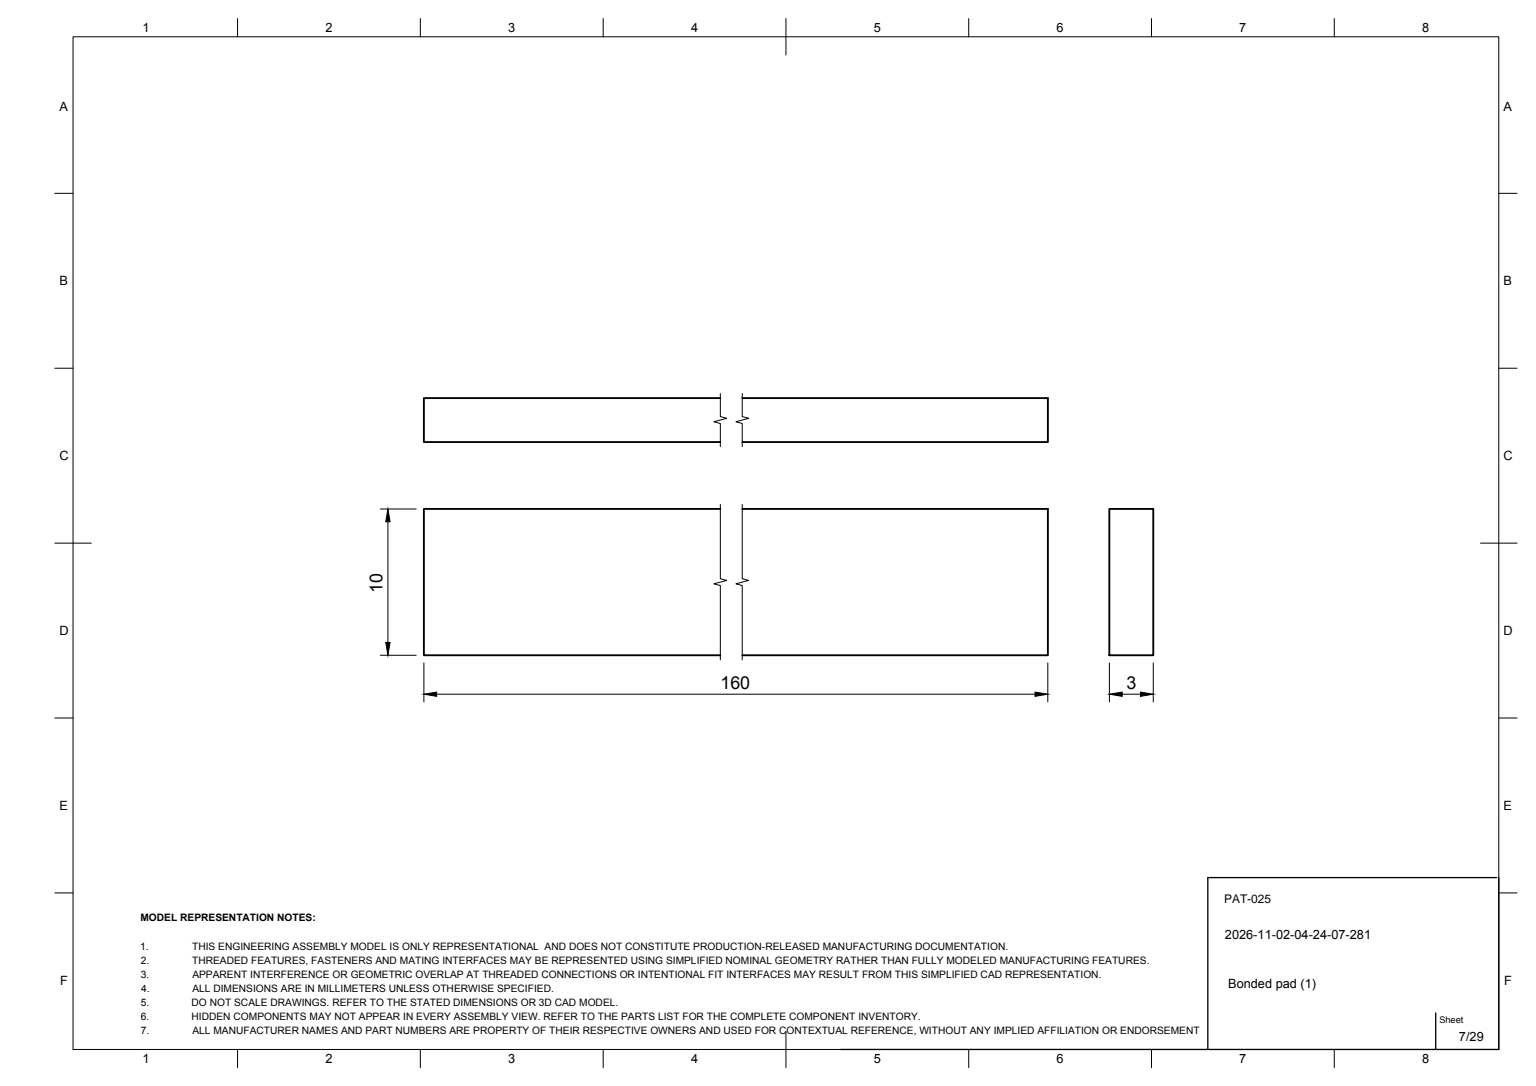
ISO-10303-21;
HEADER;
/* Generated by software containing ST-Developer
 * from STEP Tools, Inc. (www.steptools.com) 
 */

FILE_DESCRIPTION(
/* description */ ('Counter shaft with two pulleys and keyed hub'),
/* implementation_level */ '2;1');

FILE_NAME(
/* name */ 'Bonded pad (1).step',
/* time_stamp */ '2026-10-27T10:46:10-07:00',
/* author */ (''),
/* organization */ (''),
/* preprocessor_version */ 'ST-DEVELOPER v20.2',
/* originating_system */ 'Autodesk Translation Framework v15.17.0.0',
/* authorisation */ '');

FILE_SCHEMA (('AUTOMOTIVE_DESIGN { 1 0 10303 214 3 1 1 }'));
ENDSEC;

DATA;
#10=MECHANICAL_DESIGN_GEOMETRIC_PRESENTATION_REPRESENTATION('',(#292),#10821);
#242=SHAPE_REPRESENTATION_RELATIONSHIP('SRR','None',#10928,#267);
#267=ADVANCED_BREP_SHAPE_REPRESENTATION('',(#318),#10796);
#292=STYLED_ITEM('',(#11149),#318);
#318=MANIFOLD_SOLID_BREP('Body1',#5575);
#443=PLANE('',#5906);
#444=PLANE('',#5907);
#445=PLANE('',#5908);
#446=PLANE('',#5909);
#447=PLANE('',#5910);
#448=PLANE('',#5911);
#604=FACE_OUTER_BOUND('',#926,.T.);
#605=FACE_OUTER_BOUND('',#927,.T.);
#606=FACE_OUTER_BOUND('',#928,.T.);
#607=FACE_OUTER_BOUND('',#929,.T.);
#608=FACE_OUTER_BOUND('',#930,.T.);
#609=FACE_OUTER_BOUND('',#931,.T.);
#926=EDGE_LOOP('',(#3701,#3702,#3703,#3704));
#927=EDGE_LOOP('',(#3705,#3706,#3707,#3708));
#928=EDGE_LOOP('',(#3709,#3710,#3711,#3712));
#929=EDGE_LOOP('',(#3713,#3714,#3715,#3716));
#930=EDGE_LOOP('',(#3717,#3718,#3719,#3720));
#931=EDGE_LOOP('',(#3721,#3722,#3723,#3724));
#1335=LINE('',#8396,#1724);
#1336=LINE('',#8398,#1725);
#1337=LINE('',#8400,#1726);
#1338=LINE('',#8401,#1727);
#1339=LINE('',#8404,#1728);
#1340=LINE('',#8406,#1729);
#1341=LINE('',#8407,#1730);
#1342=LINE('',#8410,#1731);
#1343=LINE('',#8412,#1732);
#1344=LINE('',#8413,#1733);
#1345=LINE('',#8415,#1734);
#1346=LINE('',#8416,#1735);
#1724=VECTOR('',#6647,1.);
#1725=VECTOR('',#6648,1.);
#1726=VECTOR('',#6649,1.);
#1727=VECTOR('',#6650,1.);
#1728=VECTOR('',#6653,1.);
#1729=VECTOR('',#6654,1.);
#1730=VECTOR('',#6655,1.);
#1731=VECTOR('',#6658,1.);
#1732=VECTOR('',#6659,1.);
#1733=VECTOR('',#6660,1.);
#1734=VECTOR('',#6663,1.);
#1735=VECTOR('',#6664,1.);
#2408=VERTEX_POINT('',#8394);
#2409=VERTEX_POINT('',#8395);
#2410=VERTEX_POINT('',#8397);
#2411=VERTEX_POINT('',#8399);
#2412=VERTEX_POINT('',#8403);
#2413=VERTEX_POINT('',#8405);
#2414=VERTEX_POINT('',#8409);
#2415=VERTEX_POINT('',#8411);
#2923=EDGE_CURVE('',#2408,#2409,#1335,.T.);
#2924=EDGE_CURVE('',#2409,#2410,#1336,.T.);
#2925=EDGE_CURVE('',#2411,#2410,#1337,.T.);
#2926=EDGE_CURVE('',#2408,#2411,#1338,.T.);
#2927=EDGE_CURVE('',#2412,#2408,#1339,.T.);
#2928=EDGE_CURVE('',#2413,#2411,#1340,.T.);
#2929=EDGE_CURVE('',#2412,#2413,#1341,.T.);
#2930=EDGE_CURVE('',#2414,#2412,#1342,.T.);
#2931=EDGE_CURVE('',#2415,#2413,#1343,.T.);
#2932=EDGE_CURVE('',#2414,#2415,#1344,.T.);
#2933=EDGE_CURVE('',#2409,#2414,#1345,.T.);
#2934=EDGE_CURVE('',#2410,#2415,#1346,.T.);
#3701=ORIENTED_EDGE('',*,*,#2923,.T.);
#3702=ORIENTED_EDGE('',*,*,#2924,.T.);
#3703=ORIENTED_EDGE('',*,*,#2925,.F.);
#3704=ORIENTED_EDGE('',*,*,#2926,.F.);
#3705=ORIENTED_EDGE('',*,*,#2927,.T.);
#3706=ORIENTED_EDGE('',*,*,#2926,.T.);
#3707=ORIENTED_EDGE('',*,*,#2928,.F.);
#3708=ORIENTED_EDGE('',*,*,#2929,.F.);
#3709=ORIENTED_EDGE('',*,*,#2930,.T.);
#3710=ORIENTED_EDGE('',*,*,#2929,.T.);
#3711=ORIENTED_EDGE('',*,*,#2931,.F.);
#3712=ORIENTED_EDGE('',*,*,#2932,.F.);
#3713=ORIENTED_EDGE('',*,*,#2933,.T.);
#3714=ORIENTED_EDGE('',*,*,#2932,.T.);
#3715=ORIENTED_EDGE('',*,*,#2934,.F.);
#3716=ORIENTED_EDGE('',*,*,#2924,.F.);
#3717=ORIENTED_EDGE('',*,*,#2934,.T.);
#3718=ORIENTED_EDGE('',*,*,#2931,.T.);
#3719=ORIENTED_EDGE('',*,*,#2928,.T.);
#3720=ORIENTED_EDGE('',*,*,#2925,.T.);
#3721=ORIENTED_EDGE('',*,*,#2933,.F.);
#3722=ORIENTED_EDGE('',*,*,#2923,.F.);
#3723=ORIENTED_EDGE('',*,*,#2927,.F.);
#3724=ORIENTED_EDGE('',*,*,#2930,.F.);
#5275=ADVANCED_FACE('',(#604),#443,.T.);
#5276=ADVANCED_FACE('',(#605),#444,.T.);
#5277=ADVANCED_FACE('',(#606),#445,.T.);
#5278=ADVANCED_FACE('',(#607),#446,.T.);
#5279=ADVANCED_FACE('',(#608),#447,.T.);
#5280=ADVANCED_FACE('',(#609),#448,.F.);
#5575=CLOSED_SHELL('',(#5275,#5276,#5277,#5278,#5279,#5280));
#5905=AXIS2_PLACEMENT_3D('',#8392,#6643,#6644);
#5906=AXIS2_PLACEMENT_3D('',#8393,#6645,#6646);
#5907=AXIS2_PLACEMENT_3D('',#8402,#6651,#6652);
#5908=AXIS2_PLACEMENT_3D('',#8408,#6656,#6657);
#5909=AXIS2_PLACEMENT_3D('',#8414,#6661,#6662);
#5910=AXIS2_PLACEMENT_3D('',#8417,#6665,#6666);
#5911=AXIS2_PLACEMENT_3D('',#8418,#6667,#6668);
#6643=DIRECTION('axis',(0.,0.,1.));
#6644=DIRECTION('refdir',(1.,0.,0.));
#6645=DIRECTION('center_axis',(0.,1.,0.));
#6646=DIRECTION('ref_axis',(-1.,0.,0.));
#6647=DIRECTION('',(-1.,0.,0.));
#6648=DIRECTION('',(0.,0.,1.));
#6649=DIRECTION('',(-1.,0.,0.));
#6650=DIRECTION('',(0.,0.,1.));
#6651=DIRECTION('center_axis',(1.,0.,0.));
#6652=DIRECTION('ref_axis',(0.,1.,0.));
#6653=DIRECTION('',(0.,1.,0.));
#6654=DIRECTION('',(0.,1.,0.));
#6655=DIRECTION('',(0.,0.,1.));
#6656=DIRECTION('center_axis',(0.,-1.,0.));
#6657=DIRECTION('ref_axis',(1.,0.,0.));
#6658=DIRECTION('',(1.,0.,0.));
#6659=DIRECTION('',(1.,0.,0.));
#6660=DIRECTION('',(0.,0.,1.));
#6661=DIRECTION('center_axis',(-1.,0.,0.));
#6662=DIRECTION('ref_axis',(0.,-1.,0.));
#6663=DIRECTION('',(0.,-1.,0.));
#6664=DIRECTION('',(0.,-1.,0.));
#6665=DIRECTION('center_axis',(0.,0.,1.));
#6666=DIRECTION('ref_axis',(1.,0.,0.));
#6667=DIRECTION('center_axis',(0.,0.,1.));
#6668=DIRECTION('ref_axis',(1.,0.,0.));
#8392=CARTESIAN_POINT('',(0.,0.,0.));
#8393=CARTESIAN_POINT('Origin',(8.,29.,-0.3));
#8394=CARTESIAN_POINT('',(8.,29.,-0.3));
#8395=CARTESIAN_POINT('',(-8.,29.,-0.3));
#8396=CARTESIAN_POINT('',(8.,29.,-0.3));
#8397=CARTESIAN_POINT('',(-8.,29.,0.));
#8398=CARTESIAN_POINT('',(-8.,29.,-0.3));
#8399=CARTESIAN_POINT('',(8.,29.,0.));
#8400=CARTESIAN_POINT('',(8.,29.,0.));
#8401=CARTESIAN_POINT('',(8.,29.,-0.3));
#8402=CARTESIAN_POINT('Origin',(8.,28.,-0.3));
#8403=CARTESIAN_POINT('',(8.,28.,-0.3));
#8404=CARTESIAN_POINT('',(8.,28.,-0.3));
#8405=CARTESIAN_POINT('',(8.,28.,0.));
#8406=CARTESIAN_POINT('',(8.,28.,0.));
#8407=CARTESIAN_POINT('',(8.,28.,-0.3));
#8408=CARTESIAN_POINT('Origin',(-8.,28.,-0.3));
#8409=CARTESIAN_POINT('',(-8.,28.,-0.3));
#8410=CARTESIAN_POINT('',(-8.,28.,-0.3));
#8411=CARTESIAN_POINT('',(-8.,28.,0.));
#8412=CARTESIAN_POINT('',(-8.,28.,0.));
#8413=CARTESIAN_POINT('',(-8.,28.,-0.3));
#8414=CARTESIAN_POINT('Origin',(-8.,29.,-0.3));
#8415=CARTESIAN_POINT('',(-8.,29.,-0.3));
#8416=CARTESIAN_POINT('',(-8.,29.,0.));
#8417=CARTESIAN_POINT('Origin',(0.,28.5,0.));
#8418=CARTESIAN_POINT('Origin',(0.,28.5,-0.3));
#10766=UNCERTAINTY_MEASURE_WITH_UNIT(LENGTH_MEASURE(0.001),#10822,
'DISTANCE_ACCURACY_VALUE',
'Maximum model space distance between geometric entities at asserted c
onnectivities');
#10791=UNCERTAINTY_MEASURE_WITH_UNIT(LENGTH_MEASURE(0.001),#10822,
'DISTANCE_ACCURACY_VALUE',
'Maximum model space distance between geometric entities at asserted c
onnectivities');
#10796=(
GEOMETRIC_REPRESENTATION_CONTEXT(3)
GLOBAL_UNCERTAINTY_ASSIGNED_CONTEXT((#10766))
GLOBAL_UNIT_ASSIGNED_CONTEXT((#10822,#10824,#10825))
REPRESENTATION_CONTEXT('','3D')
);
#10821=(
GEOMETRIC_REPRESENTATION_CONTEXT(3)
GLOBAL_UNCERTAINTY_ASSIGNED_CONTEXT((#10791))
GLOBAL_UNIT_ASSIGNED_CONTEXT((#10822,#10824,#10825))
REPRESENTATION_CONTEXT('','3D')
);
#10822=(
LENGTH_UNIT()
NAMED_UNIT(*)
SI_UNIT(.CENTI.,.METRE.)
);
#10824=(
NAMED_UNIT(*)
PLANE_ANGLE_UNIT()
SI_UNIT($,.RADIAN.)
);
#10825=(
NAMED_UNIT(*)
SI_UNIT($,.STERADIAN.)
SOLID_ANGLE_UNIT()
);
#10830=SHAPE_DEFINITION_REPRESENTATION(#10859,#10928);
#10859=PRODUCT_DEFINITION_SHAPE('',$,#10958);
#10928=SHAPE_REPRESENTATION('',(#5905),#10796);
#10953=PRODUCT_DEFINITION_CONTEXT('part definition',#11042,'design');
#10958=PRODUCT_DEFINITION('Bonded pad (1)','Bonded pad (1)',#10987,#10953);
#10987=PRODUCT_DEFINITION_FORMATION('',$,#11048);
#11042=APPLICATION_CONTEXT(
'Core Data for Automotive Mechanical Design Process');
#11043=PRODUCT_CONTEXT('part definition',#11042,'mechanical');
#11048=PRODUCT('Bonded pad (1)','Bonded pad (1)','Bonded pad (1)',(#11043));
#11143=COLOUR_RGB('Off White',0.89,0.88,0.83);
#11144=FILL_AREA_STYLE_COLOUR('',#11143);
#11145=FILL_AREA_STYLE('',(#11144));
#11146=SURFACE_STYLE_FILL_AREA(#11145);
#11147=SURFACE_SIDE_STYLE('',(#11146));
#11148=SURFACE_STYLE_USAGE(.BOTH.,#11147);
#11149=PRESENTATION_STYLE_ASSIGNMENT((#11148));
ENDSEC;
END-ISO-10303-21;
